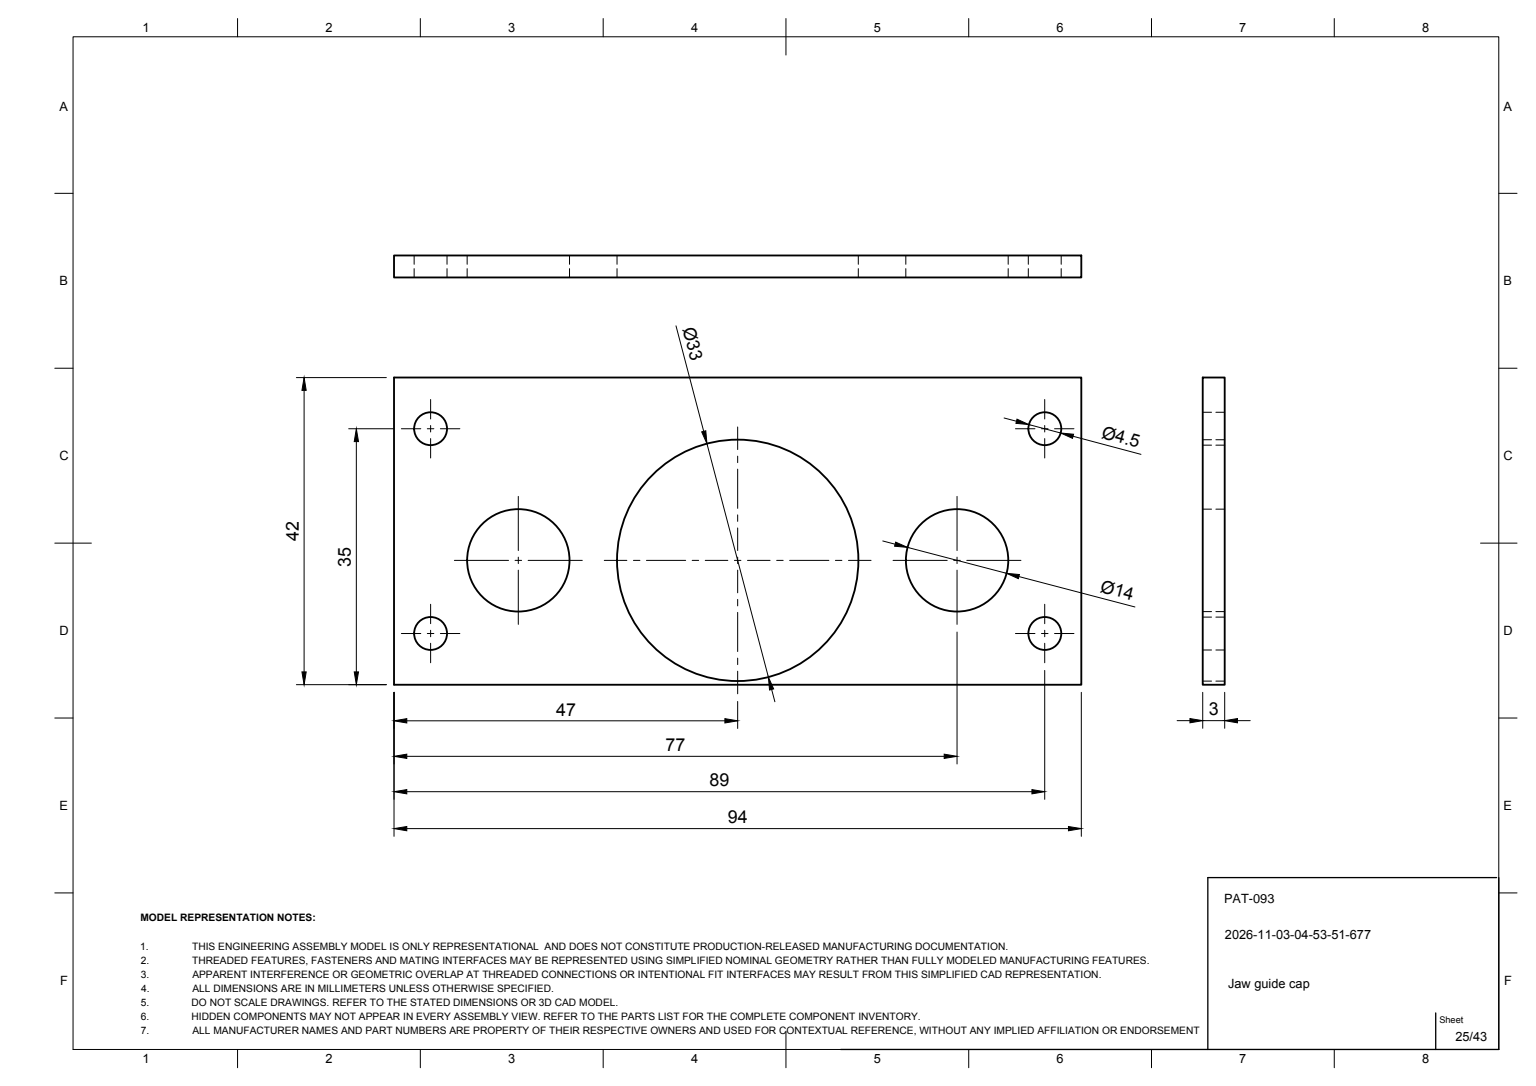
ISO-10303-21;
HEADER;
/* Generated by software containing ST-Developer
 * from STEP Tools, Inc. (www.steptools.com) 
 */

FILE_DESCRIPTION(
/* description */ ('Self-centering screw clamp'),
/* implementation_level */ '2;1');

FILE_NAME(
/* name */ 'Jaw guide cap.step',
/* time_stamp */ '2026-10-28T03:25:31-07:00',
/* author */ (''),
/* organization */ (''),
/* preprocessor_version */ 'ST-DEVELOPER v20.2',
/* originating_system */ 'Autodesk Translation Framework v15.17.0.0',
/* authorisation */ '');

FILE_SCHEMA (('AUTOMOTIVE_DESIGN { 1 0 10303 214 3 1 1 }'));
ENDSEC;

DATA;
#10=MECHANICAL_DESIGN_GEOMETRIC_PRESENTATION_REPRESENTATION('',(#651),#16799);
#562=SHAPE_REPRESENTATION_RELATIONSHIP('SRR','None',#17037,#603);
#603=ADVANCED_BREP_SHAPE_REPRESENTATION('',(#699),#16775);
#651=STYLED_ITEM('',(#17312),#699);
#699=MANIFOLD_SOLID_BREP('Body1',#9102);
#871=FACE_BOUND('',#2193,.T.);
#872=FACE_BOUND('',#2194,.T.);
#873=FACE_BOUND('',#2195,.T.);
#874=FACE_BOUND('',#2196,.T.);
#875=FACE_BOUND('',#2197,.T.);
#876=FACE_BOUND('',#2198,.T.);
#877=FACE_BOUND('',#2199,.T.);
#878=FACE_BOUND('',#2202,.T.);
#879=FACE_BOUND('',#2203,.T.);
#880=FACE_BOUND('',#2204,.T.);
#881=FACE_BOUND('',#2205,.T.);
#882=FACE_BOUND('',#2206,.T.);
#883=FACE_BOUND('',#2207,.T.);
#884=FACE_BOUND('',#2208,.T.);
#1134=PLANE('',#10157);
#1135=PLANE('',#10158);
#1136=PLANE('',#10159);
#1137=PLANE('',#10160);
#1138=PLANE('',#10161);
#1139=PLANE('',#10162);
#1527=FACE_OUTER_BOUND('',#2184,.T.);
#1528=FACE_OUTER_BOUND('',#2185,.T.);
#1529=FACE_OUTER_BOUND('',#2186,.T.);
#1530=FACE_OUTER_BOUND('',#2187,.T.);
#1531=FACE_OUTER_BOUND('',#2188,.T.);
#1532=FACE_OUTER_BOUND('',#2189,.T.);
#1533=FACE_OUTER_BOUND('',#2190,.T.);
#1534=FACE_OUTER_BOUND('',#2191,.T.);
#1535=FACE_OUTER_BOUND('',#2192,.T.);
#1536=FACE_OUTER_BOUND('',#2200,.T.);
#1537=FACE_OUTER_BOUND('',#2201,.T.);
#1538=FACE_OUTER_BOUND('',#2209,.T.);
#1539=FACE_OUTER_BOUND('',#2210,.T.);
#2184=EDGE_LOOP('',(#7293,#7294,#7295,#7296));
#2185=EDGE_LOOP('',(#7297,#7298,#7299,#7300));
#2186=EDGE_LOOP('',(#7301,#7302,#7303,#7304));
#2187=EDGE_LOOP('',(#7305,#7306,#7307,#7308));
#2188=EDGE_LOOP('',(#7309,#7310,#7311,#7312));
#2189=EDGE_LOOP('',(#7313,#7314,#7315,#7316));
#2190=EDGE_LOOP('',(#7317,#7318,#7319,#7320));
#2191=EDGE_LOOP('',(#7321,#7322,#7323,#7324));
#2192=EDGE_LOOP('',(#7325,#7326,#7327,#7328));
#2193=EDGE_LOOP('',(#7329));
#2194=EDGE_LOOP('',(#7330));
#2195=EDGE_LOOP('',(#7331));
#2196=EDGE_LOOP('',(#7332));
#2197=EDGE_LOOP('',(#7333));
#2198=EDGE_LOOP('',(#7334));
#2199=EDGE_LOOP('',(#7335));
#2200=EDGE_LOOP('',(#7336,#7337,#7338,#7339));
#2201=EDGE_LOOP('',(#7340,#7341,#7342,#7343));
#2202=EDGE_LOOP('',(#7344));
#2203=EDGE_LOOP('',(#7345));
#2204=EDGE_LOOP('',(#7346));
#2205=EDGE_LOOP('',(#7347));
#2206=EDGE_LOOP('',(#7348));
#2207=EDGE_LOOP('',(#7349));
#2208=EDGE_LOOP('',(#7350));
#2209=EDGE_LOOP('',(#7351,#7352,#7353,#7354));
#2210=EDGE_LOOP('',(#7355,#7356,#7357,#7358));
#2867=LINE('',#15324,#3440);
#2868=LINE('',#15330,#3441);
#2869=LINE('',#15336,#3442);
#2870=LINE('',#15342,#3443);
#2871=LINE('',#15348,#3444);
#2872=LINE('',#15354,#3445);
#2873=LINE('',#15360,#3446);
#2874=LINE('',#15365,#3447);
#2875=LINE('',#15367,#3448);
#2876=LINE('',#15369,#3449);
#2877=LINE('',#15370,#3450);
#2878=LINE('',#15373,#3451);
#2879=LINE('',#15375,#3452);
#2880=LINE('',#15376,#3453);
#2881=LINE('',#15379,#3454);
#2882=LINE('',#15381,#3455);
#2883=LINE('',#15382,#3456);
#2884=LINE('',#15384,#3457);
#2885=LINE('',#15385,#3458);
#3440=VECTOR('',#12164,0.225);
#3441=VECTOR('',#12171,0.225);
#3442=VECTOR('',#12178,0.225);
#3443=VECTOR('',#12185,0.225);
#3444=VECTOR('',#12192,1.65);
#3445=VECTOR('',#12199,0.7);
#3446=VECTOR('',#12206,0.7);
#3447=VECTOR('',#12211,1.);
#3448=VECTOR('',#12212,1.);
#3449=VECTOR('',#12213,1.);
#3450=VECTOR('',#12214,1.);
#3451=VECTOR('',#12217,1.);
#3452=VECTOR('',#12218,1.);
#3453=VECTOR('',#12219,1.);
#3454=VECTOR('',#12222,1.);
#3455=VECTOR('',#12223,1.);
#3456=VECTOR('',#12224,1.);
#3457=VECTOR('',#12227,1.);
#3458=VECTOR('',#12228,1.);
#3998=CIRCLE('',#10137,0.225);
#3999=CIRCLE('',#10138,0.225);
#4000=CIRCLE('',#10140,0.225);
#4001=CIRCLE('',#10141,0.225);
#4002=CIRCLE('',#10143,0.225);
#4003=CIRCLE('',#10144,0.225);
#4004=CIRCLE('',#10146,0.225);
#4005=CIRCLE('',#10147,0.225);
#4006=CIRCLE('',#10149,1.65);
#4007=CIRCLE('',#10150,1.65);
#4008=CIRCLE('',#10152,0.7);
#4009=CIRCLE('',#10153,0.7);
#4010=CIRCLE('',#10155,0.7);
#4011=CIRCLE('',#10156,0.7);
#4625=VERTEX_POINT('',#15321);
#4626=VERTEX_POINT('',#15323);
#4627=VERTEX_POINT('',#15327);
#4628=VERTEX_POINT('',#15329);
#4629=VERTEX_POINT('',#15333);
#4630=VERTEX_POINT('',#15335);
#4631=VERTEX_POINT('',#15339);
#4632=VERTEX_POINT('',#15341);
#4633=VERTEX_POINT('',#15345);
#4634=VERTEX_POINT('',#15347);
#4635=VERTEX_POINT('',#15351);
#4636=VERTEX_POINT('',#15353);
#4637=VERTEX_POINT('',#15357);
#4638=VERTEX_POINT('',#15359);
#4639=VERTEX_POINT('',#15363);
#4640=VERTEX_POINT('',#15364);
#4641=VERTEX_POINT('',#15366);
#4642=VERTEX_POINT('',#15368);
#4643=VERTEX_POINT('',#15372);
#4644=VERTEX_POINT('',#15374);
#4645=VERTEX_POINT('',#15378);
#4646=VERTEX_POINT('',#15380);
#5571=EDGE_CURVE('',#4625,#4625,#3998,.T.);
#5572=EDGE_CURVE('',#4625,#4626,#2867,.T.);
#5573=EDGE_CURVE('',#4626,#4626,#3999,.T.);
#5574=EDGE_CURVE('',#4627,#4627,#4000,.T.);
#5575=EDGE_CURVE('',#4627,#4628,#2868,.T.);
#5576=EDGE_CURVE('',#4628,#4628,#4001,.T.);
#5577=EDGE_CURVE('',#4629,#4629,#4002,.T.);
#5578=EDGE_CURVE('',#4629,#4630,#2869,.T.);
#5579=EDGE_CURVE('',#4630,#4630,#4003,.T.);
#5580=EDGE_CURVE('',#4631,#4631,#4004,.T.);
#5581=EDGE_CURVE('',#4631,#4632,#2870,.T.);
#5582=EDGE_CURVE('',#4632,#4632,#4005,.T.);
#5583=EDGE_CURVE('',#4633,#4633,#4006,.T.);
#5584=EDGE_CURVE('',#4633,#4634,#2871,.T.);
#5585=EDGE_CURVE('',#4634,#4634,#4007,.T.);
#5586=EDGE_CURVE('',#4635,#4635,#4008,.T.);
#5587=EDGE_CURVE('',#4635,#4636,#2872,.T.);
#5588=EDGE_CURVE('',#4636,#4636,#4009,.T.);
#5589=EDGE_CURVE('',#4637,#4637,#4010,.T.);
#5590=EDGE_CURVE('',#4637,#4638,#2873,.T.);
#5591=EDGE_CURVE('',#4638,#4638,#4011,.T.);
#5592=EDGE_CURVE('',#4639,#4640,#2874,.T.);
#5593=EDGE_CURVE('',#4640,#4641,#2875,.T.);
#5594=EDGE_CURVE('',#4642,#4641,#2876,.T.);
#5595=EDGE_CURVE('',#4639,#4642,#2877,.T.);
#5596=EDGE_CURVE('',#4643,#4639,#2878,.T.);
#5597=EDGE_CURVE('',#4644,#4642,#2879,.T.);
#5598=EDGE_CURVE('',#4643,#4644,#2880,.T.);
#5599=EDGE_CURVE('',#4645,#4643,#2881,.T.);
#5600=EDGE_CURVE('',#4646,#4644,#2882,.T.);
#5601=EDGE_CURVE('',#4645,#4646,#2883,.T.);
#5602=EDGE_CURVE('',#4640,#4645,#2884,.T.);
#5603=EDGE_CURVE('',#4641,#4646,#2885,.T.);
#7293=ORIENTED_EDGE('',*,*,#5571,.F.);
#7294=ORIENTED_EDGE('',*,*,#5572,.T.);
#7295=ORIENTED_EDGE('',*,*,#5573,.F.);
#7296=ORIENTED_EDGE('',*,*,#5572,.F.);
#7297=ORIENTED_EDGE('',*,*,#5574,.F.);
#7298=ORIENTED_EDGE('',*,*,#5575,.T.);
#7299=ORIENTED_EDGE('',*,*,#5576,.F.);
#7300=ORIENTED_EDGE('',*,*,#5575,.F.);
#7301=ORIENTED_EDGE('',*,*,#5577,.F.);
#7302=ORIENTED_EDGE('',*,*,#5578,.T.);
#7303=ORIENTED_EDGE('',*,*,#5579,.F.);
#7304=ORIENTED_EDGE('',*,*,#5578,.F.);
#7305=ORIENTED_EDGE('',*,*,#5580,.F.);
#7306=ORIENTED_EDGE('',*,*,#5581,.T.);
#7307=ORIENTED_EDGE('',*,*,#5582,.F.);
#7308=ORIENTED_EDGE('',*,*,#5581,.F.);
#7309=ORIENTED_EDGE('',*,*,#5583,.F.);
#7310=ORIENTED_EDGE('',*,*,#5584,.T.);
#7311=ORIENTED_EDGE('',*,*,#5585,.F.);
#7312=ORIENTED_EDGE('',*,*,#5584,.F.);
#7313=ORIENTED_EDGE('',*,*,#5586,.F.);
#7314=ORIENTED_EDGE('',*,*,#5587,.T.);
#7315=ORIENTED_EDGE('',*,*,#5588,.F.);
#7316=ORIENTED_EDGE('',*,*,#5587,.F.);
#7317=ORIENTED_EDGE('',*,*,#5589,.F.);
#7318=ORIENTED_EDGE('',*,*,#5590,.T.);
#7319=ORIENTED_EDGE('',*,*,#5591,.F.);
#7320=ORIENTED_EDGE('',*,*,#5590,.F.);
#7321=ORIENTED_EDGE('',*,*,#5592,.T.);
#7322=ORIENTED_EDGE('',*,*,#5593,.T.);
#7323=ORIENTED_EDGE('',*,*,#5594,.F.);
#7324=ORIENTED_EDGE('',*,*,#5595,.F.);
#7325=ORIENTED_EDGE('',*,*,#5596,.T.);
#7326=ORIENTED_EDGE('',*,*,#5595,.T.);
#7327=ORIENTED_EDGE('',*,*,#5597,.F.);
#7328=ORIENTED_EDGE('',*,*,#5598,.F.);
#7329=ORIENTED_EDGE('',*,*,#5591,.T.);
#7330=ORIENTED_EDGE('',*,*,#5588,.T.);
#7331=ORIENTED_EDGE('',*,*,#5585,.T.);
#7332=ORIENTED_EDGE('',*,*,#5582,.T.);
#7333=ORIENTED_EDGE('',*,*,#5579,.T.);
#7334=ORIENTED_EDGE('',*,*,#5576,.T.);
#7335=ORIENTED_EDGE('',*,*,#5573,.T.);
#7336=ORIENTED_EDGE('',*,*,#5599,.T.);
#7337=ORIENTED_EDGE('',*,*,#5598,.T.);
#7338=ORIENTED_EDGE('',*,*,#5600,.F.);
#7339=ORIENTED_EDGE('',*,*,#5601,.F.);
#7340=ORIENTED_EDGE('',*,*,#5602,.T.);
#7341=ORIENTED_EDGE('',*,*,#5601,.T.);
#7342=ORIENTED_EDGE('',*,*,#5603,.F.);
#7343=ORIENTED_EDGE('',*,*,#5593,.F.);
#7344=ORIENTED_EDGE('',*,*,#5589,.T.);
#7345=ORIENTED_EDGE('',*,*,#5586,.T.);
#7346=ORIENTED_EDGE('',*,*,#5583,.T.);
#7347=ORIENTED_EDGE('',*,*,#5580,.T.);
#7348=ORIENTED_EDGE('',*,*,#5577,.T.);
#7349=ORIENTED_EDGE('',*,*,#5574,.T.);
#7350=ORIENTED_EDGE('',*,*,#5571,.T.);
#7351=ORIENTED_EDGE('',*,*,#5603,.T.);
#7352=ORIENTED_EDGE('',*,*,#5600,.T.);
#7353=ORIENTED_EDGE('',*,*,#5597,.T.);
#7354=ORIENTED_EDGE('',*,*,#5594,.T.);
#7355=ORIENTED_EDGE('',*,*,#5602,.F.);
#7356=ORIENTED_EDGE('',*,*,#5592,.F.);
#7357=ORIENTED_EDGE('',*,*,#5596,.F.);
#7358=ORIENTED_EDGE('',*,*,#5599,.F.);
#8469=CYLINDRICAL_SURFACE('',#10136,0.225);
#8470=CYLINDRICAL_SURFACE('',#10139,0.225);
#8471=CYLINDRICAL_SURFACE('',#10142,0.225);
#8472=CYLINDRICAL_SURFACE('',#10145,0.225);
#8473=CYLINDRICAL_SURFACE('',#10148,1.65);
#8474=CYLINDRICAL_SURFACE('',#10151,0.7);
#8475=CYLINDRICAL_SURFACE('',#10154,0.7);
#8825=ADVANCED_FACE('',(#1527),#8469,.F.);
#8826=ADVANCED_FACE('',(#1528),#8470,.F.);
#8827=ADVANCED_FACE('',(#1529),#8471,.F.);
#8828=ADVANCED_FACE('',(#1530),#8472,.F.);
#8829=ADVANCED_FACE('',(#1531),#8473,.F.);
#8830=ADVANCED_FACE('',(#1532),#8474,.F.);
#8831=ADVANCED_FACE('',(#1533),#8475,.F.);
#8832=ADVANCED_FACE('',(#1534),#1134,.T.);
#8833=ADVANCED_FACE('',(#1535,#871,#872,#873,#874,#875,#876,#877),#1135,
 .T.);
#8834=ADVANCED_FACE('',(#1536),#1136,.T.);
#8835=ADVANCED_FACE('',(#1537,#878,#879,#880,#881,#882,#883,#884),#1137,
 .T.);
#8836=ADVANCED_FACE('',(#1538),#1138,.T.);
#8837=ADVANCED_FACE('',(#1539),#1139,.F.);
#9102=CLOSED_SHELL('',(#8825,#8826,#8827,#8828,#8829,#8830,#8831,#8832,
#8833,#8834,#8835,#8836,#8837));
#10135=AXIS2_PLACEMENT_3D('',#15319,#12158,#12159);
#10136=AXIS2_PLACEMENT_3D('',#15320,#12160,#12161);
#10137=AXIS2_PLACEMENT_3D('',#15322,#12162,#12163);
#10138=AXIS2_PLACEMENT_3D('',#15325,#12165,#12166);
#10139=AXIS2_PLACEMENT_3D('',#15326,#12167,#12168);
#10140=AXIS2_PLACEMENT_3D('',#15328,#12169,#12170);
#10141=AXIS2_PLACEMENT_3D('',#15331,#12172,#12173);
#10142=AXIS2_PLACEMENT_3D('',#15332,#12174,#12175);
#10143=AXIS2_PLACEMENT_3D('',#15334,#12176,#12177);
#10144=AXIS2_PLACEMENT_3D('',#15337,#12179,#12180);
#10145=AXIS2_PLACEMENT_3D('',#15338,#12181,#12182);
#10146=AXIS2_PLACEMENT_3D('',#15340,#12183,#12184);
#10147=AXIS2_PLACEMENT_3D('',#15343,#12186,#12187);
#10148=AXIS2_PLACEMENT_3D('',#15344,#12188,#12189);
#10149=AXIS2_PLACEMENT_3D('',#15346,#12190,#12191);
#10150=AXIS2_PLACEMENT_3D('',#15349,#12193,#12194);
#10151=AXIS2_PLACEMENT_3D('',#15350,#12195,#12196);
#10152=AXIS2_PLACEMENT_3D('',#15352,#12197,#12198);
#10153=AXIS2_PLACEMENT_3D('',#15355,#12200,#12201);
#10154=AXIS2_PLACEMENT_3D('',#15356,#12202,#12203);
#10155=AXIS2_PLACEMENT_3D('',#15358,#12204,#12205);
#10156=AXIS2_PLACEMENT_3D('',#15361,#12207,#12208);
#10157=AXIS2_PLACEMENT_3D('',#15362,#12209,#12210);
#10158=AXIS2_PLACEMENT_3D('',#15371,#12215,#12216);
#10159=AXIS2_PLACEMENT_3D('',#15377,#12220,#12221);
#10160=AXIS2_PLACEMENT_3D('',#15383,#12225,#12226);
#10161=AXIS2_PLACEMENT_3D('',#15386,#12229,#12230);
#10162=AXIS2_PLACEMENT_3D('',#15387,#12231,#12232);
#12158=DIRECTION('axis',(0.,0.,1.));
#12159=DIRECTION('refdir',(1.,0.,0.));
#12160=DIRECTION('center_axis',(1.,0.,0.));
#12161=DIRECTION('ref_axis',(0.,0.,-1.));
#12162=DIRECTION('center_axis',(1.,0.,0.));
#12163=DIRECTION('ref_axis',(0.,0.,-1.));
#12164=DIRECTION('',(1.,0.,0.));
#12165=DIRECTION('center_axis',(-1.,0.,0.));
#12166=DIRECTION('ref_axis',(0.,0.,-1.));
#12167=DIRECTION('center_axis',(1.,0.,0.));
#12168=DIRECTION('ref_axis',(0.,0.,-1.));
#12169=DIRECTION('center_axis',(1.,0.,0.));
#12170=DIRECTION('ref_axis',(0.,0.,-1.));
#12171=DIRECTION('',(1.,0.,0.));
#12172=DIRECTION('center_axis',(-1.,0.,0.));
#12173=DIRECTION('ref_axis',(0.,0.,-1.));
#12174=DIRECTION('center_axis',(1.,0.,0.));
#12175=DIRECTION('ref_axis',(0.,0.,-1.));
#12176=DIRECTION('center_axis',(1.,0.,0.));
#12177=DIRECTION('ref_axis',(0.,0.,-1.));
#12178=DIRECTION('',(1.,0.,0.));
#12179=DIRECTION('center_axis',(-1.,0.,0.));
#12180=DIRECTION('ref_axis',(0.,0.,-1.));
#12181=DIRECTION('center_axis',(1.,0.,0.));
#12182=DIRECTION('ref_axis',(0.,0.,-1.));
#12183=DIRECTION('center_axis',(1.,0.,0.));
#12184=DIRECTION('ref_axis',(0.,0.,-1.));
#12185=DIRECTION('',(1.,0.,0.));
#12186=DIRECTION('center_axis',(-1.,0.,0.));
#12187=DIRECTION('ref_axis',(0.,0.,-1.));
#12188=DIRECTION('center_axis',(1.,0.,0.));
#12189=DIRECTION('ref_axis',(0.,0.,-1.));
#12190=DIRECTION('center_axis',(1.,0.,0.));
#12191=DIRECTION('ref_axis',(0.,0.,-1.));
#12192=DIRECTION('',(1.,0.,0.));
#12193=DIRECTION('center_axis',(-1.,0.,0.));
#12194=DIRECTION('ref_axis',(0.,0.,-1.));
#12195=DIRECTION('center_axis',(1.,0.,0.));
#12196=DIRECTION('ref_axis',(0.,0.,-1.));
#12197=DIRECTION('center_axis',(1.,0.,0.));
#12198=DIRECTION('ref_axis',(0.,0.,-1.));
#12199=DIRECTION('',(1.,0.,0.));
#12200=DIRECTION('center_axis',(-1.,0.,0.));
#12201=DIRECTION('ref_axis',(0.,0.,-1.));
#12202=DIRECTION('center_axis',(1.,0.,0.));
#12203=DIRECTION('ref_axis',(0.,0.,-1.));
#12204=DIRECTION('center_axis',(1.,0.,0.));
#12205=DIRECTION('ref_axis',(0.,0.,-1.));
#12206=DIRECTION('',(1.,0.,0.));
#12207=DIRECTION('center_axis',(-1.,0.,0.));
#12208=DIRECTION('ref_axis',(0.,0.,-1.));
#12209=DIRECTION('center_axis',(0.,1.,0.));
#12210=DIRECTION('ref_axis',(-1.,0.,0.));
#12211=DIRECTION('',(-1.,0.,0.));
#12212=DIRECTION('',(0.,0.,1.));
#12213=DIRECTION('',(-1.,0.,0.));
#12214=DIRECTION('',(0.,0.,1.));
#12215=DIRECTION('center_axis',(1.,0.,0.));
#12216=DIRECTION('ref_axis',(0.,1.,0.));
#12217=DIRECTION('',(0.,1.,0.));
#12218=DIRECTION('',(0.,1.,0.));
#12219=DIRECTION('',(0.,0.,1.));
#12220=DIRECTION('center_axis',(0.,-1.,0.));
#12221=DIRECTION('ref_axis',(1.,0.,0.));
#12222=DIRECTION('',(1.,0.,0.));
#12223=DIRECTION('',(1.,0.,0.));
#12224=DIRECTION('',(0.,0.,1.));
#12225=DIRECTION('center_axis',(-1.,0.,0.));
#12226=DIRECTION('ref_axis',(0.,-1.,0.));
#12227=DIRECTION('',(0.,-1.,0.));
#12228=DIRECTION('',(0.,-1.,0.));
#12229=DIRECTION('center_axis',(0.,0.,1.));
#12230=DIRECTION('ref_axis',(1.,0.,0.));
#12231=DIRECTION('center_axis',(0.,0.,1.));
#12232=DIRECTION('ref_axis',(1.,0.,0.));
#15319=CARTESIAN_POINT('',(0.,0.,0.));
#15320=CARTESIAN_POINT('Origin',(-8.9,4.2,3.));
#15321=CARTESIAN_POINT('',(-8.8,4.2,3.225));
#15322=CARTESIAN_POINT('Origin',(-8.8,4.2,3.));
#15323=CARTESIAN_POINT('',(-8.5,4.2,3.225));
#15324=CARTESIAN_POINT('',(-8.9,4.2,3.225));
#15325=CARTESIAN_POINT('Origin',(-8.5,4.2,3.));
#15326=CARTESIAN_POINT('Origin',(-8.9,-4.2,5.8));
#15327=CARTESIAN_POINT('',(-8.8,-4.2,6.025));
#15328=CARTESIAN_POINT('Origin',(-8.8,-4.2,5.8));
#15329=CARTESIAN_POINT('',(-8.5,-4.2,6.025));
#15330=CARTESIAN_POINT('',(-8.9,-4.2,6.025));
#15331=CARTESIAN_POINT('Origin',(-8.5,-4.2,5.8));
#15332=CARTESIAN_POINT('Origin',(-8.9,-4.2,3.));
#15333=CARTESIAN_POINT('',(-8.8,-4.2,3.225));
#15334=CARTESIAN_POINT('Origin',(-8.8,-4.2,3.));
#15335=CARTESIAN_POINT('',(-8.5,-4.2,3.225));
#15336=CARTESIAN_POINT('',(-8.9,-4.2,3.225));
#15337=CARTESIAN_POINT('Origin',(-8.5,-4.2,3.));
#15338=CARTESIAN_POINT('Origin',(-8.9,4.2,5.8));
#15339=CARTESIAN_POINT('',(-8.8,4.2,6.025));
#15340=CARTESIAN_POINT('Origin',(-8.8,4.2,5.8));
#15341=CARTESIAN_POINT('',(-8.5,4.2,6.025));
#15342=CARTESIAN_POINT('',(-8.9,4.2,6.025));
#15343=CARTESIAN_POINT('Origin',(-8.5,4.2,5.8));
#15344=CARTESIAN_POINT('Origin',(-8.9,0.,4.));
#15345=CARTESIAN_POINT('',(-8.8,-2.02066721859313E-16,5.65));
#15346=CARTESIAN_POINT('Origin',(-8.8,0.,4.));
#15347=CARTESIAN_POINT('',(-8.5,2.02066721859313E-16,5.65));
#15348=CARTESIAN_POINT('',(-8.9,-2.02066721859313E-16,5.65));
#15349=CARTESIAN_POINT('Origin',(-8.5,0.,4.));
#15350=CARTESIAN_POINT('Origin',(-8.9,-3.,4.));
#15351=CARTESIAN_POINT('',(-8.8,-3.,4.7));
#15352=CARTESIAN_POINT('Origin',(-8.8,-3.,4.));
#15353=CARTESIAN_POINT('',(-8.5,-3.,4.7));
#15354=CARTESIAN_POINT('',(-8.9,-3.,4.7));
#15355=CARTESIAN_POINT('Origin',(-8.5,-3.,4.));
#15356=CARTESIAN_POINT('Origin',(-8.9,3.,4.));
#15357=CARTESIAN_POINT('',(-8.8,3.,4.7));
#15358=CARTESIAN_POINT('Origin',(-8.8,3.,4.));
#15359=CARTESIAN_POINT('',(-8.5,3.,4.7));
#15360=CARTESIAN_POINT('',(-8.9,3.,4.7));
#15361=CARTESIAN_POINT('Origin',(-8.5,3.,4.));
#15362=CARTESIAN_POINT('Origin',(-8.5,4.7,2.3));
#15363=CARTESIAN_POINT('',(-8.5,4.7,2.3));
#15364=CARTESIAN_POINT('',(-8.8,4.7,2.3));
#15365=CARTESIAN_POINT('',(-8.5,4.7,2.3));
#15366=CARTESIAN_POINT('',(-8.8,4.7,6.5));
#15367=CARTESIAN_POINT('',(-8.8,4.7,2.3));
#15368=CARTESIAN_POINT('',(-8.5,4.7,6.5));
#15369=CARTESIAN_POINT('',(-8.5,4.7,6.5));
#15370=CARTESIAN_POINT('',(-8.5,4.7,2.3));
#15371=CARTESIAN_POINT('Origin',(-8.5,-4.7,2.3));
#15372=CARTESIAN_POINT('',(-8.5,-4.7,2.3));
#15373=CARTESIAN_POINT('',(-8.5,-4.7,2.3));
#15374=CARTESIAN_POINT('',(-8.5,-4.7,6.5));
#15375=CARTESIAN_POINT('',(-8.5,-4.7,6.5));
#15376=CARTESIAN_POINT('',(-8.5,-4.7,2.3));
#15377=CARTESIAN_POINT('Origin',(-8.8,-4.7,2.3));
#15378=CARTESIAN_POINT('',(-8.8,-4.7,2.3));
#15379=CARTESIAN_POINT('',(-8.8,-4.7,2.3));
#15380=CARTESIAN_POINT('',(-8.8,-4.7,6.5));
#15381=CARTESIAN_POINT('',(-8.8,-4.7,6.5));
#15382=CARTESIAN_POINT('',(-8.8,-4.7,2.3));
#15383=CARTESIAN_POINT('Origin',(-8.8,4.7,2.3));
#15384=CARTESIAN_POINT('',(-8.8,4.7,2.3));
#15385=CARTESIAN_POINT('',(-8.8,4.7,6.5));
#15386=CARTESIAN_POINT('Origin',(-8.65,0.,6.5));
#15387=CARTESIAN_POINT('Origin',(-8.65,0.,2.3));
#16726=UNCERTAINTY_MEASURE_WITH_UNIT(LENGTH_MEASURE(0.001),#16800,
'DISTANCE_ACCURACY_VALUE',
'Maximum model space distance between geometric entities at asserted c
onnectivities');
#16750=UNCERTAINTY_MEASURE_WITH_UNIT(LENGTH_MEASURE(0.001),#16800,
'DISTANCE_ACCURACY_VALUE',
'Maximum model space distance between geometric entities at asserted c
onnectivities');
#16775=(
GEOMETRIC_REPRESENTATION_CONTEXT(3)
GLOBAL_UNCERTAINTY_ASSIGNED_CONTEXT((#16726))
GLOBAL_UNIT_ASSIGNED_CONTEXT((#16800,#16802,#16803))
REPRESENTATION_CONTEXT('','3D')
);
#16799=(
GEOMETRIC_REPRESENTATION_CONTEXT(3)
GLOBAL_UNCERTAINTY_ASSIGNED_CONTEXT((#16750))
GLOBAL_UNIT_ASSIGNED_CONTEXT((#16800,#16802,#16803))
REPRESENTATION_CONTEXT('','3D')
);
#16800=(
LENGTH_UNIT()
NAMED_UNIT(*)
SI_UNIT(.CENTI.,.METRE.)
);
#16802=(
NAMED_UNIT(*)
PLANE_ANGLE_UNIT()
SI_UNIT($,.RADIAN.)
);
#16803=(
NAMED_UNIT(*)
SI_UNIT($,.STERADIAN.)
SOLID_ANGLE_UNIT()
);
#16828=SHAPE_DEFINITION_REPRESENTATION(#16881,#17037);
#16881=PRODUCT_DEFINITION_SHAPE('',$,#17086);
#17037=SHAPE_REPRESENTATION('',(#10135),#16775);
#17061=PRODUCT_DEFINITION_CONTEXT('part definition',#17207,'design');
#17086=PRODUCT_DEFINITION('Jaw guide cap','Jaw guide cap',#17134,#17061);
#17134=PRODUCT_DEFINITION_FORMATION('',$,#17233);
#17207=APPLICATION_CONTEXT(
'Core Data for Automotive Mechanical Design Process');
#17208=PRODUCT_CONTEXT('part definition',#17207,'mechanical');
#17233=PRODUCT('Jaw guide cap','Jaw guide cap','Jaw guide cap',(#17208));
#17306=COLOUR_RGB('Light Blue',0.38,0.62,0.78);
#17307=FILL_AREA_STYLE_COLOUR('',#17306);
#17308=FILL_AREA_STYLE('',(#17307));
#17309=SURFACE_STYLE_FILL_AREA(#17308);
#17310=SURFACE_SIDE_STYLE('',(#17309));
#17311=SURFACE_STYLE_USAGE(.BOTH.,#17310);
#17312=PRESENTATION_STYLE_ASSIGNMENT((#17311));
ENDSEC;
END-ISO-10303-21;
